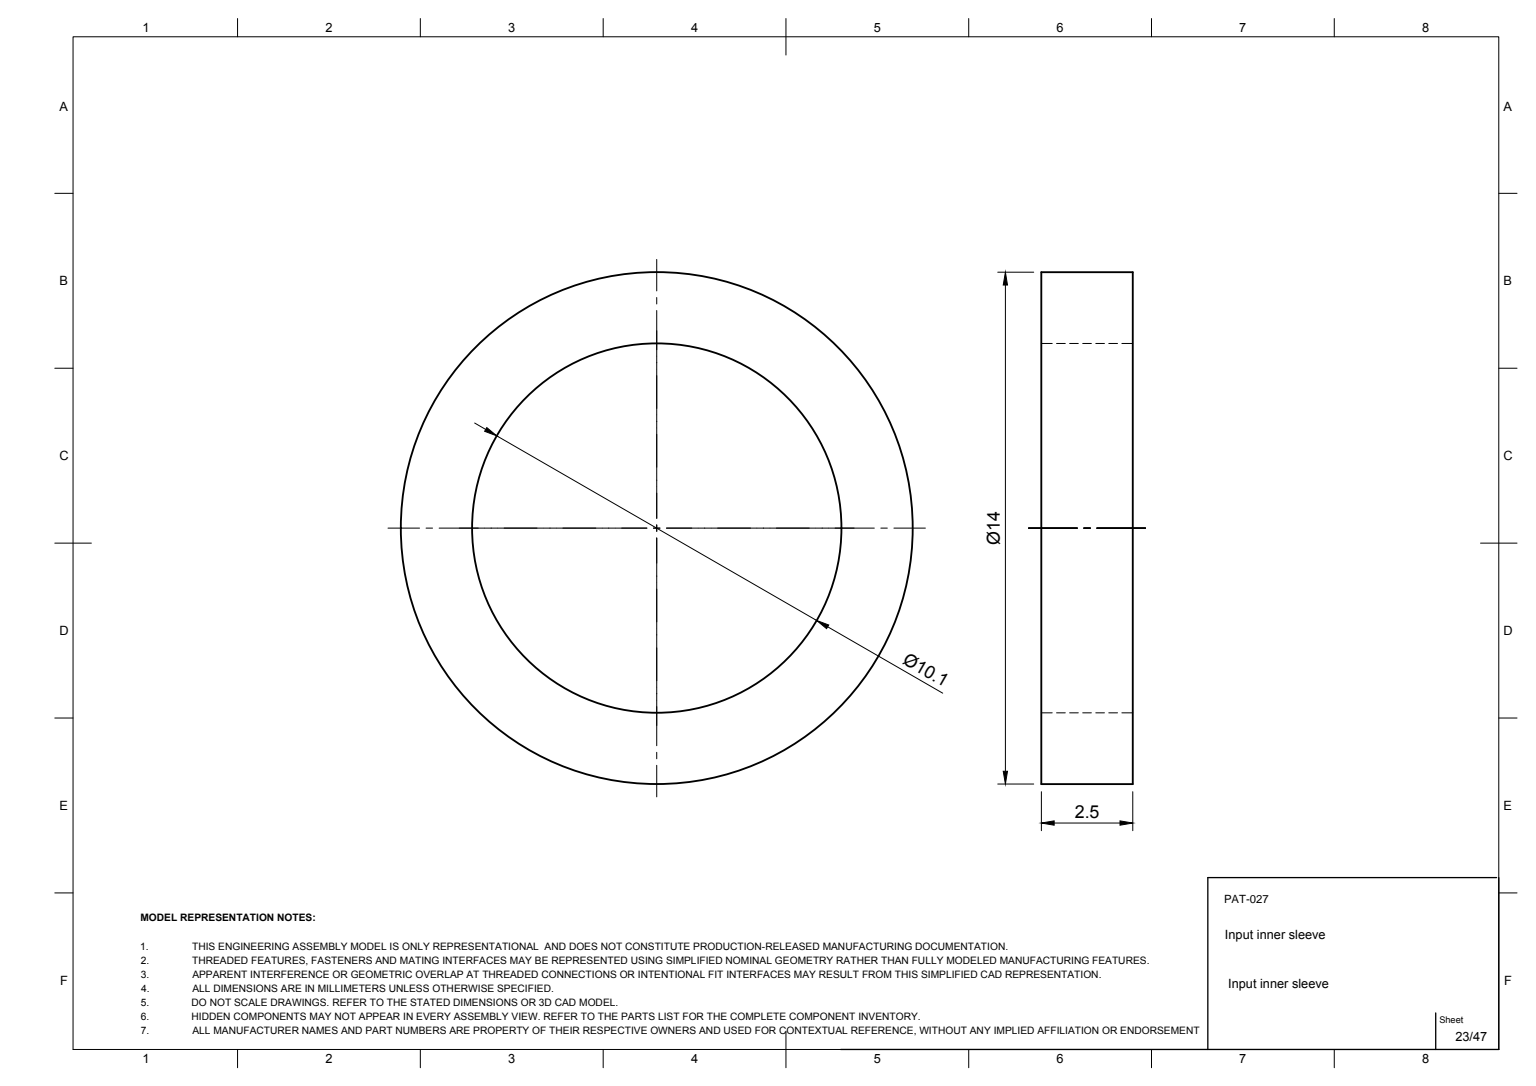
ISO-10303-21;
HEADER;
/* Generated by software containing ST-Developer
 * from STEP Tools, Inc. (www.steptools.com) 
 */

FILE_DESCRIPTION(
/* description */ ('Crank-driven oscillating fan base (mechanism only)'),

/* implementation_level */ '2;1');

FILE_NAME(
/* name */ 'Input inner sleeve.step',
/* time_stamp */ '2026-10-28T03:25:00-07:00',
/* author */ (''),
/* organization */ (''),
/* preprocessor_version */ 'ST-DEVELOPER v20.2',
/* originating_system */ 'Autodesk Translation Framework v15.17.0.0',
/* authorisation */ '');

FILE_SCHEMA (('AUTOMOTIVE_DESIGN { 1 0 10303 214 3 1 1 }'));
ENDSEC;

DATA;
#10=MECHANICAL_DESIGN_GEOMETRIC_PRESENTATION_REPRESENTATION('',(#460),#11916);
#372=SHAPE_REPRESENTATION_RELATIONSHIP('SRR','None',#12098,#412);
#412=ADVANCED_BREP_SHAPE_REPRESENTATION('',(#507),#11889);
#460=STYLED_ITEM('',(#12361),#507);
#507=MANIFOLD_SOLID_BREP('Body1',#6091);
#622=FACE_BOUND('',#1546,.T.);
#623=FACE_BOUND('',#1548,.T.);
#778=PLANE('',#7001);
#779=PLANE('',#7002);
#1076=FACE_OUTER_BOUND('',#1543,.T.);
#1077=FACE_OUTER_BOUND('',#1544,.T.);
#1078=FACE_OUTER_BOUND('',#1545,.T.);
#1079=FACE_OUTER_BOUND('',#1547,.T.);
#1543=EDGE_LOOP('',(#4870,#4871,#4872,#4873));
#1544=EDGE_LOOP('',(#4874,#4875,#4876,#4877));
#1545=EDGE_LOOP('',(#4878));
#1546=EDGE_LOOP('',(#4879));
#1547=EDGE_LOOP('',(#4880));
#1548=EDGE_LOOP('',(#4881));
#1952=LINE('',#10819,#2285);
#1953=LINE('',#10825,#2286);
#2285=VECTOR('',#8441,0.505);
#2286=VECTOR('',#8448,0.7);
#2685=CIRCLE('',#6996,0.505);
#2686=CIRCLE('',#6997,0.505);
#2687=CIRCLE('',#6999,0.7);
#2688=CIRCLE('',#7000,0.7);
#3106=VERTEX_POINT('',#10816);
#3107=VERTEX_POINT('',#10818);
#3108=VERTEX_POINT('',#10822);
#3109=VERTEX_POINT('',#10824);
#3730=EDGE_CURVE('',#3106,#3106,#2685,.T.);
#3731=EDGE_CURVE('',#3106,#3107,#1952,.T.);
#3732=EDGE_CURVE('',#3107,#3107,#2686,.T.);
#3733=EDGE_CURVE('',#3108,#3108,#2687,.T.);
#3734=EDGE_CURVE('',#3108,#3109,#1953,.T.);
#3735=EDGE_CURVE('',#3109,#3109,#2688,.T.);
#4870=ORIENTED_EDGE('',*,*,#3730,.F.);
#4871=ORIENTED_EDGE('',*,*,#3731,.T.);
#4872=ORIENTED_EDGE('',*,*,#3732,.T.);
#4873=ORIENTED_EDGE('',*,*,#3731,.F.);
#4874=ORIENTED_EDGE('',*,*,#3733,.F.);
#4875=ORIENTED_EDGE('',*,*,#3734,.T.);
#4876=ORIENTED_EDGE('',*,*,#3735,.T.);
#4877=ORIENTED_EDGE('',*,*,#3734,.F.);
#4878=ORIENTED_EDGE('',*,*,#3733,.T.);
#4879=ORIENTED_EDGE('',*,*,#3730,.T.);
#4880=ORIENTED_EDGE('',*,*,#3735,.F.);
#4881=ORIENTED_EDGE('',*,*,#3732,.F.);
#5625=CYLINDRICAL_SURFACE('',#6995,0.505);
#5626=CYLINDRICAL_SURFACE('',#6998,0.7);
#5882=ADVANCED_FACE('',(#1076),#5625,.F.);
#5883=ADVANCED_FACE('',(#1077),#5626,.T.);
#5884=ADVANCED_FACE('',(#1078,#622),#778,.T.);
#5885=ADVANCED_FACE('',(#1079,#623),#779,.F.);
#6091=CLOSED_SHELL('',(#5882,#5883,#5884,#5885));
#6994=AXIS2_PLACEMENT_3D('',#10814,#8435,#8436);
#6995=AXIS2_PLACEMENT_3D('',#10815,#8437,#8438);
#6996=AXIS2_PLACEMENT_3D('',#10817,#8439,#8440);
#6997=AXIS2_PLACEMENT_3D('',#10820,#8442,#8443);
#6998=AXIS2_PLACEMENT_3D('',#10821,#8444,#8445);
#6999=AXIS2_PLACEMENT_3D('',#10823,#8446,#8447);
#7000=AXIS2_PLACEMENT_3D('',#10826,#8449,#8450);
#7001=AXIS2_PLACEMENT_3D('',#10827,#8451,#8452);
#7002=AXIS2_PLACEMENT_3D('',#10828,#8453,#8454);
#8435=DIRECTION('axis',(0.,0.,1.));
#8436=DIRECTION('refdir',(1.,0.,0.));
#8437=DIRECTION('center_axis',(0.,0.,1.));
#8438=DIRECTION('ref_axis',(1.,0.,0.));
#8439=DIRECTION('center_axis',(0.,0.,-1.));
#8440=DIRECTION('ref_axis',(1.,0.,0.));
#8441=DIRECTION('',(0.,0.,-1.));
#8442=DIRECTION('center_axis',(0.,0.,-1.));
#8443=DIRECTION('ref_axis',(1.,0.,0.));
#8444=DIRECTION('center_axis',(0.,0.,1.));
#8445=DIRECTION('ref_axis',(1.,0.,0.));
#8446=DIRECTION('center_axis',(0.,0.,1.));
#8447=DIRECTION('ref_axis',(1.,0.,0.));
#8448=DIRECTION('',(0.,0.,-1.));
#8449=DIRECTION('center_axis',(0.,0.,1.));
#8450=DIRECTION('ref_axis',(1.,0.,0.));
#8451=DIRECTION('center_axis',(0.,0.,1.));
#8452=DIRECTION('ref_axis',(1.,0.,0.));
#8453=DIRECTION('center_axis',(0.,0.,1.));
#8454=DIRECTION('ref_axis',(1.,0.,0.));
#10814=CARTESIAN_POINT('',(0.,0.,0.));
#10815=CARTESIAN_POINT('Origin',(0.,0.,1.8));
#10816=CARTESIAN_POINT('',(-0.505,-6.18446633569413E-17,2.05));
#10817=CARTESIAN_POINT('Origin',(0.,0.,2.05));
#10818=CARTESIAN_POINT('',(-0.505,-6.18446633569413E-17,1.8));
#10819=CARTESIAN_POINT('',(-0.505,-6.18446633569413E-17,1.8));
#10820=CARTESIAN_POINT('Origin',(0.,0.,1.8));
#10821=CARTESIAN_POINT('Origin',(0.,0.,1.8));
#10822=CARTESIAN_POINT('',(-0.7,-8.57252759403147E-17,2.05));
#10823=CARTESIAN_POINT('Origin',(0.,0.,2.05));
#10824=CARTESIAN_POINT('',(-0.7,-8.57252759403147E-17,1.8));
#10825=CARTESIAN_POINT('',(-0.7,-8.57252759403147E-17,1.8));
#10826=CARTESIAN_POINT('Origin',(0.,0.,1.8));
#10827=CARTESIAN_POINT('Origin',(0.,0.,2.05));
#10828=CARTESIAN_POINT('Origin',(0.,0.,1.8));
#11842=UNCERTAINTY_MEASURE_WITH_UNIT(LENGTH_MEASURE(0.001),#11917,
'DISTANCE_ACCURACY_VALUE',
'Maximum model space distance between geometric entities at asserted c
onnectivities');
#11869=UNCERTAINTY_MEASURE_WITH_UNIT(LENGTH_MEASURE(0.001),#11917,
'DISTANCE_ACCURACY_VALUE',
'Maximum model space distance between geometric entities at asserted c
onnectivities');
#11889=(
GEOMETRIC_REPRESENTATION_CONTEXT(3)
GLOBAL_UNCERTAINTY_ASSIGNED_CONTEXT((#11842))
GLOBAL_UNIT_ASSIGNED_CONTEXT((#11917,#11919,#11920))
REPRESENTATION_CONTEXT('','3D')
);
#11916=(
GEOMETRIC_REPRESENTATION_CONTEXT(3)
GLOBAL_UNCERTAINTY_ASSIGNED_CONTEXT((#11869))
GLOBAL_UNIT_ASSIGNED_CONTEXT((#11917,#11919,#11920))
REPRESENTATION_CONTEXT('','3D')
);
#11917=(
LENGTH_UNIT()
NAMED_UNIT(*)
SI_UNIT(.CENTI.,.METRE.)
);
#11919=(
NAMED_UNIT(*)
PLANE_ANGLE_UNIT()
SI_UNIT($,.RADIAN.)
);
#11920=(
NAMED_UNIT(*)
SI_UNIT($,.STERADIAN.)
SOLID_ANGLE_UNIT()
);
#11940=SHAPE_DEFINITION_REPRESENTATION(#11991,#12098);
#11991=PRODUCT_DEFINITION_SHAPE('',$,#12145);
#12098=SHAPE_REPRESENTATION('',(#6994),#11889);
#12125=PRODUCT_DEFINITION_CONTEXT('part definition',#12265,'design');
#12145=PRODUCT_DEFINITION('Input inner sleeve','Input inner sleeve',#12191,
#12125);
#12191=PRODUCT_DEFINITION_FORMATION('',$,#12286);
#12265=APPLICATION_CONTEXT(
'Core Data for Automotive Mechanical Design Process');
#12266=PRODUCT_CONTEXT('part definition',#12265,'mechanical');
#12286=PRODUCT('Input inner sleeve','Input inner sleeve',
'Input inner sleeve',(#12266));
#12355=COLOUR_RGB('Light Blue',0.38,0.62,0.78);
#12356=FILL_AREA_STYLE_COLOUR('',#12355);
#12357=FILL_AREA_STYLE('',(#12356));
#12358=SURFACE_STYLE_FILL_AREA(#12357);
#12359=SURFACE_SIDE_STYLE('',(#12358));
#12360=SURFACE_STYLE_USAGE(.BOTH.,#12359);
#12361=PRESENTATION_STYLE_ASSIGNMENT((#12360));
ENDSEC;
END-ISO-10303-21;
